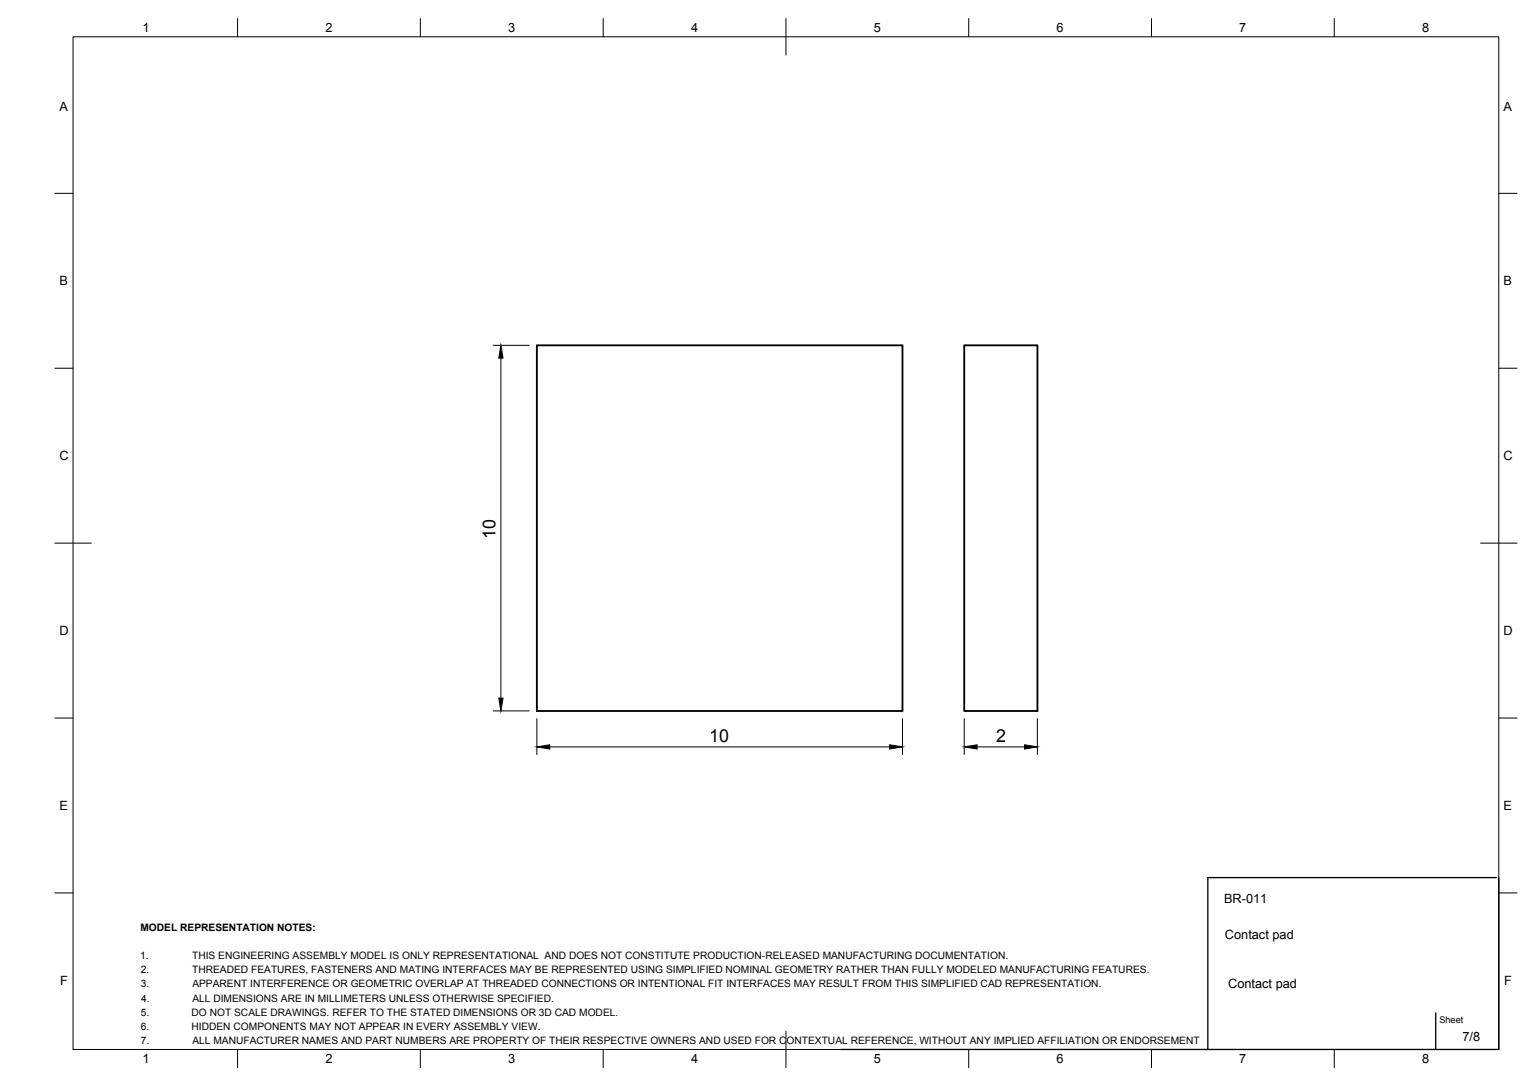
ISO-10303-21;
HEADER;
/* Generated by software containing ST-Developer
 * from STEP Tools, Inc. (www.steptools.com) 
 */

FILE_DESCRIPTION(
/* description */ ('Independent pair of monolithic parallel-leaf compliant finger modules.
 Shared native part/module instances; external gripper actuator outsid
e scope. Whole-mm geometry,1mm webs,56mm straight span,12mm depth,32mm
 nominal contact gap. Undeformed CAD reference; material condition, el
astic range, fatigue and gripping force unassigned.'),
/* implementation_level */ '2;1');

FILE_NAME(
/* name */ 'Contact pad.step',
/* time_stamp */ '2026-11-07T22:36:16-08:00',
/* author */ (''),
/* organization */ (''),
/* preprocessor_version */ 'ST-DEVELOPER v20.2',
/* originating_system */ 'Autodesk Translation Framework v15.17.0.0',
/* authorisation */ '');

FILE_SCHEMA (('AUTOMOTIVE_DESIGN { 1 0 10303 214 3 1 1 }'));
ENDSEC;

DATA;
#10=MECHANICAL_DESIGN_GEOMETRIC_PRESENTATION_REPRESENTATION('',(#331),#13801);
#319=SHAPE_REPRESENTATION_RELATIONSHIP('SRR','None',#13837,#325);
#325=ADVANCED_BREP_SHAPE_REPRESENTATION('',(#337),#13797);
#331=STYLED_ITEM('',(#13880),#337);
#337=MANIFOLD_SOLID_BREP('Body1',#3696);
#397=PLANE('',#3926);
#398=PLANE('',#3927);
#399=PLANE('',#3928);
#400=PLANE('',#3929);
#401=PLANE('',#3930);
#402=PLANE('',#3931);
#529=FACE_OUTER_BOUND('',#750,.T.);
#530=FACE_OUTER_BOUND('',#751,.T.);
#531=FACE_OUTER_BOUND('',#752,.T.);
#532=FACE_OUTER_BOUND('',#753,.T.);
#533=FACE_OUTER_BOUND('',#754,.T.);
#534=FACE_OUTER_BOUND('',#755,.T.);
#750=EDGE_LOOP('',(#2877,#2878,#2879,#2880));
#751=EDGE_LOOP('',(#2881,#2882,#2883,#2884));
#752=EDGE_LOOP('',(#2885,#2886,#2887,#2888));
#753=EDGE_LOOP('',(#2889,#2890,#2891,#2892));
#754=EDGE_LOOP('',(#2893,#2894,#2895,#2896));
#755=EDGE_LOOP('',(#2897,#2898,#2899,#2900));
#977=LINE('',#9357,#1206);
#978=LINE('',#9359,#1207);
#979=LINE('',#9361,#1208);
#980=LINE('',#9362,#1209);
#981=LINE('',#9365,#1210);
#982=LINE('',#9367,#1211);
#983=LINE('',#9368,#1212);
#984=LINE('',#9371,#1213);
#985=LINE('',#9373,#1214);
#986=LINE('',#9374,#1215);
#987=LINE('',#9376,#1216);
#988=LINE('',#9377,#1217);
#1206=VECTOR('',#4494,10.);
#1207=VECTOR('',#4495,10.);
#1208=VECTOR('',#4496,10.);
#1209=VECTOR('',#4497,10.);
#1210=VECTOR('',#4500,10.);
#1211=VECTOR('',#4501,10.);
#1212=VECTOR('',#4502,10.);
#1213=VECTOR('',#4505,10.);
#1214=VECTOR('',#4506,10.);
#1215=VECTOR('',#4507,10.);
#1216=VECTOR('',#4510,10.);
#1217=VECTOR('',#4511,10.);
#1564=VERTEX_POINT('',#9355);
#1565=VERTEX_POINT('',#9356);
#1566=VERTEX_POINT('',#9358);
#1567=VERTEX_POINT('',#9360);
#1568=VERTEX_POINT('',#9364);
#1569=VERTEX_POINT('',#9366);
#1570=VERTEX_POINT('',#9370);
#1571=VERTEX_POINT('',#9372);
#2028=EDGE_CURVE('',#1564,#1565,#977,.T.);
#2029=EDGE_CURVE('',#1565,#1566,#978,.T.);
#2030=EDGE_CURVE('',#1567,#1566,#979,.T.);
#2031=EDGE_CURVE('',#1564,#1567,#980,.T.);
#2032=EDGE_CURVE('',#1568,#1564,#981,.T.);
#2033=EDGE_CURVE('',#1569,#1567,#982,.T.);
#2034=EDGE_CURVE('',#1568,#1569,#983,.T.);
#2035=EDGE_CURVE('',#1570,#1568,#984,.T.);
#2036=EDGE_CURVE('',#1571,#1569,#985,.T.);
#2037=EDGE_CURVE('',#1570,#1571,#986,.T.);
#2038=EDGE_CURVE('',#1565,#1570,#987,.T.);
#2039=EDGE_CURVE('',#1566,#1571,#988,.T.);
#2877=ORIENTED_EDGE('',*,*,#2028,.T.);
#2878=ORIENTED_EDGE('',*,*,#2029,.T.);
#2879=ORIENTED_EDGE('',*,*,#2030,.F.);
#2880=ORIENTED_EDGE('',*,*,#2031,.F.);
#2881=ORIENTED_EDGE('',*,*,#2032,.T.);
#2882=ORIENTED_EDGE('',*,*,#2031,.T.);
#2883=ORIENTED_EDGE('',*,*,#2033,.F.);
#2884=ORIENTED_EDGE('',*,*,#2034,.F.);
#2885=ORIENTED_EDGE('',*,*,#2035,.T.);
#2886=ORIENTED_EDGE('',*,*,#2034,.T.);
#2887=ORIENTED_EDGE('',*,*,#2036,.F.);
#2888=ORIENTED_EDGE('',*,*,#2037,.F.);
#2889=ORIENTED_EDGE('',*,*,#2038,.T.);
#2890=ORIENTED_EDGE('',*,*,#2037,.T.);
#2891=ORIENTED_EDGE('',*,*,#2039,.F.);
#2892=ORIENTED_EDGE('',*,*,#2029,.F.);
#2893=ORIENTED_EDGE('',*,*,#2039,.T.);
#2894=ORIENTED_EDGE('',*,*,#2036,.T.);
#2895=ORIENTED_EDGE('',*,*,#2033,.T.);
#2896=ORIENTED_EDGE('',*,*,#2030,.T.);
#2897=ORIENTED_EDGE('',*,*,#2038,.F.);
#2898=ORIENTED_EDGE('',*,*,#2028,.F.);
#2899=ORIENTED_EDGE('',*,*,#2032,.F.);
#2900=ORIENTED_EDGE('',*,*,#2035,.F.);
#3605=ADVANCED_FACE('',(#529),#397,.T.);
#3606=ADVANCED_FACE('',(#530),#398,.T.);
#3607=ADVANCED_FACE('',(#531),#399,.T.);
#3608=ADVANCED_FACE('',(#532),#400,.T.);
#3609=ADVANCED_FACE('',(#533),#401,.T.);
#3610=ADVANCED_FACE('',(#534),#402,.F.);
#3696=CLOSED_SHELL('',(#3605,#3606,#3607,#3608,#3609,#3610));
#3925=AXIS2_PLACEMENT_3D('',#9353,#4490,#4491);
#3926=AXIS2_PLACEMENT_3D('',#9354,#4492,#4493);
#3927=AXIS2_PLACEMENT_3D('',#9363,#4498,#4499);
#3928=AXIS2_PLACEMENT_3D('',#9369,#4503,#4504);
#3929=AXIS2_PLACEMENT_3D('',#9375,#4508,#4509);
#3930=AXIS2_PLACEMENT_3D('',#9378,#4512,#4513);
#3931=AXIS2_PLACEMENT_3D('',#9379,#4514,#4515);
#4490=DIRECTION('axis',(0.,0.,1.));
#4491=DIRECTION('refdir',(1.,0.,0.));
#4492=DIRECTION('center_axis',(0.,1.,0.));
#4493=DIRECTION('ref_axis',(-1.,0.,0.));
#4494=DIRECTION('',(-1.,0.,0.));
#4495=DIRECTION('',(0.,0.,1.));
#4496=DIRECTION('',(-1.,0.,0.));
#4497=DIRECTION('',(0.,0.,1.));
#4498=DIRECTION('center_axis',(1.,0.,0.));
#4499=DIRECTION('ref_axis',(0.,1.,0.));
#4500=DIRECTION('',(0.,1.,0.));
#4501=DIRECTION('',(0.,1.,0.));
#4502=DIRECTION('',(0.,0.,1.));
#4503=DIRECTION('center_axis',(0.,-1.,0.));
#4504=DIRECTION('ref_axis',(1.,0.,0.));
#4505=DIRECTION('',(1.,0.,0.));
#4506=DIRECTION('',(1.,0.,0.));
#4507=DIRECTION('',(0.,0.,1.));
#4508=DIRECTION('center_axis',(-1.,0.,0.));
#4509=DIRECTION('ref_axis',(0.,-1.,0.));
#4510=DIRECTION('',(0.,-1.,0.));
#4511=DIRECTION('',(0.,-1.,0.));
#4512=DIRECTION('center_axis',(0.,0.,1.));
#4513=DIRECTION('ref_axis',(1.,0.,0.));
#4514=DIRECTION('center_axis',(0.,0.,1.));
#4515=DIRECTION('ref_axis',(1.,0.,0.));
#9353=CARTESIAN_POINT('',(0.,0.,0.));
#9354=CARTESIAN_POINT('Origin',(94.,-12.,-5.));
#9355=CARTESIAN_POINT('',(94.,-12.,-5.));
#9356=CARTESIAN_POINT('',(84.,-12.,-5.));
#9357=CARTESIAN_POINT('',(94.,-12.,-5.));
#9358=CARTESIAN_POINT('',(84.,-12.,5.));
#9359=CARTESIAN_POINT('',(84.,-12.,-5.));
#9360=CARTESIAN_POINT('',(94.,-12.,5.));
#9361=CARTESIAN_POINT('',(94.,-12.,5.));
#9362=CARTESIAN_POINT('',(94.,-12.,-5.));
#9363=CARTESIAN_POINT('Origin',(94.,-14.,-5.));
#9364=CARTESIAN_POINT('',(94.,-14.,-5.));
#9365=CARTESIAN_POINT('',(94.,-14.,-5.));
#9366=CARTESIAN_POINT('',(94.,-14.,5.));
#9367=CARTESIAN_POINT('',(94.,-14.,5.));
#9368=CARTESIAN_POINT('',(94.,-14.,-5.));
#9369=CARTESIAN_POINT('Origin',(84.,-14.,-5.));
#9370=CARTESIAN_POINT('',(84.,-14.,-5.));
#9371=CARTESIAN_POINT('',(84.,-14.,-5.));
#9372=CARTESIAN_POINT('',(84.,-14.,5.));
#9373=CARTESIAN_POINT('',(84.,-14.,5.));
#9374=CARTESIAN_POINT('',(84.,-14.,-5.));
#9375=CARTESIAN_POINT('Origin',(84.,-12.,-5.));
#9376=CARTESIAN_POINT('',(84.,-12.,-5.));
#9377=CARTESIAN_POINT('',(84.,-12.,5.));
#9378=CARTESIAN_POINT('Origin',(89.,-13.,5.));
#9379=CARTESIAN_POINT('Origin',(89.,-13.,-5.));
#13788=UNCERTAINTY_MEASURE_WITH_UNIT(LENGTH_MEASURE(0.01),#13802,
'DISTANCE_ACCURACY_VALUE',
'Maximum model space distance between geometric entities at asserted c
onnectivities');
#13792=UNCERTAINTY_MEASURE_WITH_UNIT(LENGTH_MEASURE(0.01),#13802,
'DISTANCE_ACCURACY_VALUE',
'Maximum model space distance between geometric entities at asserted c
onnectivities');
#13797=(
GEOMETRIC_REPRESENTATION_CONTEXT(3)
GLOBAL_UNCERTAINTY_ASSIGNED_CONTEXT((#13788))
GLOBAL_UNIT_ASSIGNED_CONTEXT((#13802,#13804,#13805))
REPRESENTATION_CONTEXT('','3D')
);
#13801=(
GEOMETRIC_REPRESENTATION_CONTEXT(3)
GLOBAL_UNCERTAINTY_ASSIGNED_CONTEXT((#13792))
GLOBAL_UNIT_ASSIGNED_CONTEXT((#13802,#13804,#13805))
REPRESENTATION_CONTEXT('','3D')
);
#13802=(
LENGTH_UNIT()
NAMED_UNIT(*)
SI_UNIT(.MILLI.,.METRE.)
);
#13804=(
NAMED_UNIT(*)
PLANE_ANGLE_UNIT()
SI_UNIT($,.RADIAN.)
);
#13805=(
NAMED_UNIT(*)
SI_UNIT($,.STERADIAN.)
SOLID_ANGLE_UNIT()
);
#13810=SHAPE_DEFINITION_REPRESENTATION(#13818,#13837);
#13818=PRODUCT_DEFINITION_SHAPE('',$,#13846);
#13837=SHAPE_REPRESENTATION('',(#3925),#13797);
#13841=PRODUCT_DEFINITION_CONTEXT('part definition',#13867,'design');
#13846=PRODUCT_DEFINITION('Contact pad','Contact pad',#13854,#13841);
#13854=PRODUCT_DEFINITION_FORMATION('',$,#13873);
#13867=APPLICATION_CONTEXT(
'Core Data for Automotive Mechanical Design Process');
#13868=PRODUCT_CONTEXT('part definition',#13867,'mechanical');
#13873=PRODUCT('Contact pad','Contact pad',$,(#13868));
#13880=PRESENTATION_STYLE_ASSIGNMENT((#13887));
#13887=SURFACE_STYLE_USAGE(.BOTH.,#13894);
#13894=SURFACE_SIDE_STYLE('',(#13901));
#13901=SURFACE_STYLE_FILL_AREA(#13908);
#13908=FILL_AREA_STYLE('Light blue',(#13915));
#13915=FILL_AREA_STYLE_COLOUR('Light blue',#13922);
#13922=COLOUR_RGB('Light blue',0.662745098039216,0.831372549019608,0.949019607843137);
ENDSEC;
END-ISO-10303-21;
